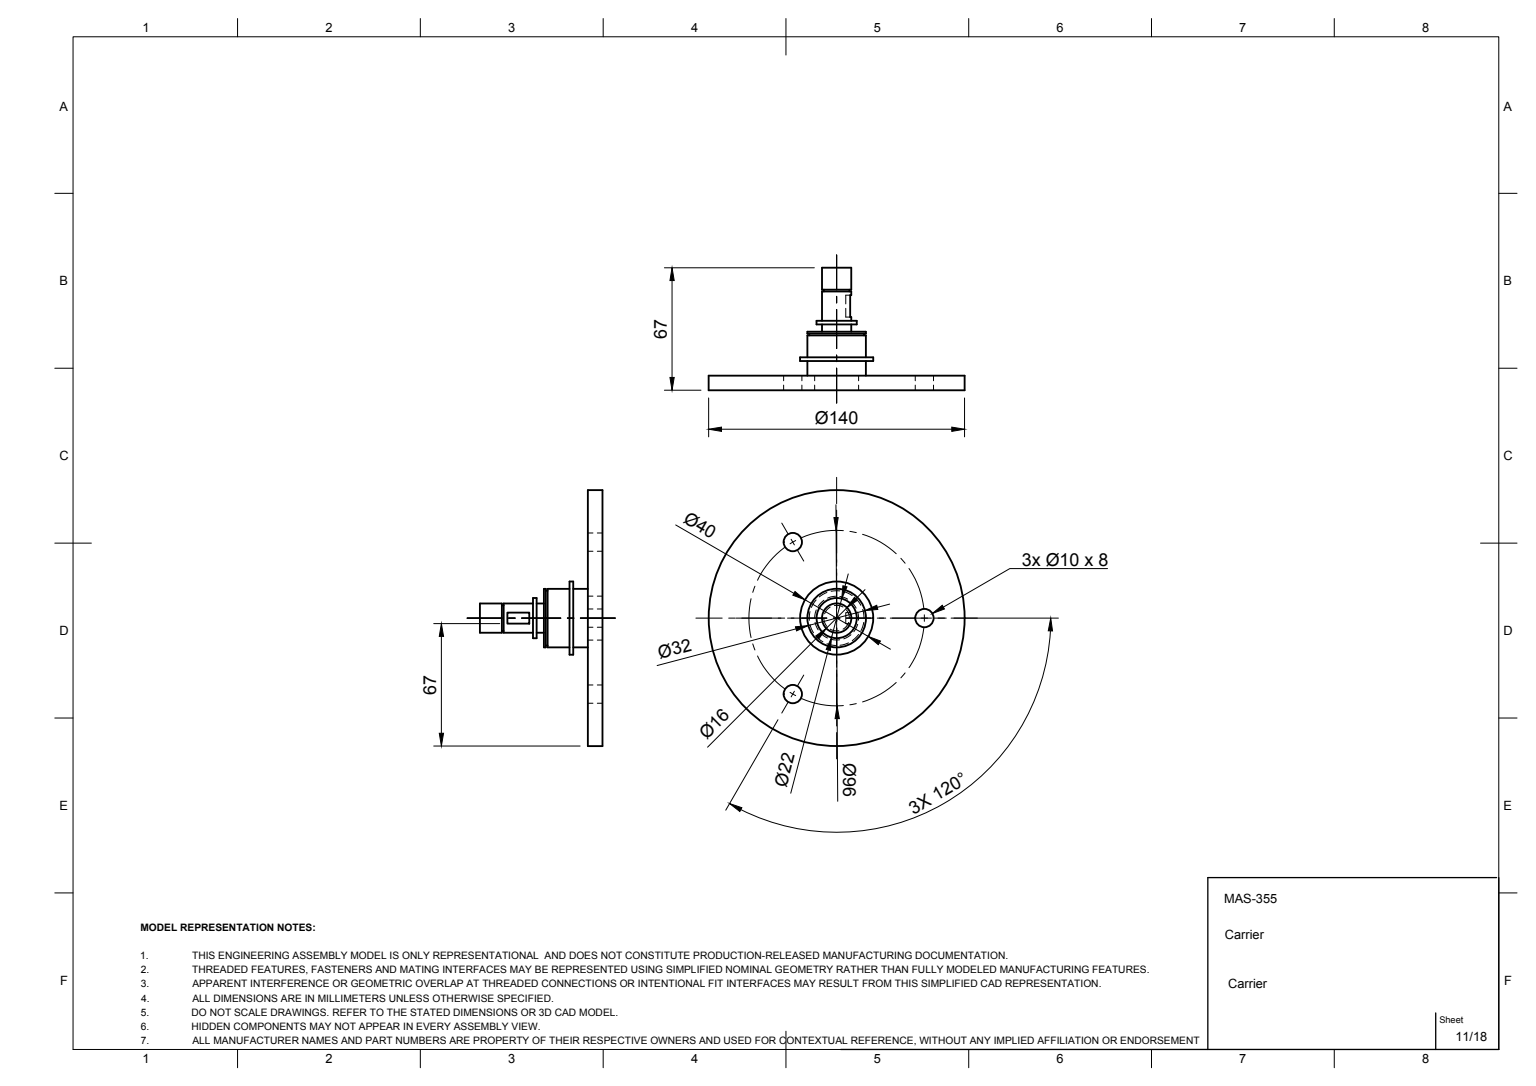
ISO-10303-21;
HEADER;
/* Generated by software containing ST-Developer
 * from STEP Tools, Inc. (www.steptools.com) 
 */

FILE_DESCRIPTION(
/* description */ ('Independent two-stage fixed-ring planetary gearbox,24/24/72 teeth,mod
ule2,20deg involutes,three planets per stage,4:1 x4:1=16:1. Native cut
-space/fillet/pattern tooth profiles derived from reusable gear blanks
; shared sun/planet/ring/carrier parts across both stages. Captured br
onze-journal input/carriers, headed retained planet pins, keyed inters
tage drive and modular keyed output interface. Native ideal gear links
; no torque, precision grade, production backlash/fits, lubrication, s
peed or life rating.'),
/* implementation_level */ '2;1');

FILE_NAME(
/* name */ 'Carrier.step',
/* time_stamp */ '2026-11-08T19:10:00-08:00',
/* author */ (''),
/* organization */ (''),
/* preprocessor_version */ 'ST-DEVELOPER v20.2',
/* originating_system */ 'Autodesk Translation Framework v15.17.0.0',
/* authorisation */ '');

FILE_SCHEMA (('AUTOMOTIVE_DESIGN { 1 0 10303 214 3 1 1 }'));
ENDSEC;

DATA;
#10=MECHANICAL_DESIGN_GEOMETRIC_PRESENTATION_REPRESENTATION('',(#1171),#259224);
#1131=SHAPE_REPRESENTATION_RELATIONSHIP('SRR','None',#259378,#1151);
#1151=ADVANCED_BREP_SHAPE_REPRESENTATION('',(#1191),#259212);
#1171=STYLED_ITEM('',(#259486),#1191);
#1191=MANIFOLD_SOLID_BREP('Body1',#25158);
#1287=FACE_BOUND('',#4341,.T.);
#1288=FACE_BOUND('',#4343,.T.);
#1289=FACE_BOUND('',#4347,.T.);
#1290=FACE_BOUND('',#4349,.T.);
#1291=FACE_BOUND('',#4355,.T.);
#1292=FACE_BOUND('',#4357,.T.);
#1293=FACE_BOUND('',#4361,.T.);
#1294=FACE_BOUND('',#4364,.T.);
#1295=FACE_BOUND('',#4366,.T.);
#1296=FACE_BOUND('',#4372,.T.);
#1297=FACE_BOUND('',#4376,.T.);
#1298=FACE_BOUND('',#4377,.T.);
#1299=FACE_BOUND('',#4378,.T.);
#1300=FACE_BOUND('',#4379,.T.);
#1301=FACE_BOUND('',#4381,.T.);
#1302=FACE_BOUND('',#4382,.T.);
#1303=FACE_BOUND('',#4383,.T.);
#1304=FACE_BOUND('',#4384,.T.);
#1637=PLANE('',#27011);
#1638=PLANE('',#27012);
#1639=PLANE('',#27014);
#1640=PLANE('',#27015);
#1641=PLANE('',#27016);
#1642=PLANE('',#27021);
#1643=PLANE('',#27023);
#1644=PLANE('',#27030);
#1645=PLANE('',#27032);
#1646=PLANE('',#27045);
#1647=PLANE('',#27048);
#1648=PLANE('',#27055);
#1649=PLANE('',#27056);
#1650=PLANE('',#27059);
#1651=PLANE('',#27065);
#1652=PLANE('',#27068);
#1653=PLANE('',#27074);
#1654=PLANE('',#27075);
#2904=FACE_OUTER_BOUND('',#4334,.T.);
#2905=FACE_OUTER_BOUND('',#4335,.T.);
#2906=FACE_OUTER_BOUND('',#4336,.T.);
#2907=FACE_OUTER_BOUND('',#4337,.T.);
#2908=FACE_OUTER_BOUND('',#4338,.T.);
#2909=FACE_OUTER_BOUND('',#4339,.T.);
#2910=FACE_OUTER_BOUND('',#4340,.T.);
#2911=FACE_OUTER_BOUND('',#4342,.T.);
#2912=FACE_OUTER_BOUND('',#4344,.T.);
#2913=FACE_OUTER_BOUND('',#4345,.T.);
#2914=FACE_OUTER_BOUND('',#4346,.T.);
#2915=FACE_OUTER_BOUND('',#4348,.T.);
#2916=FACE_OUTER_BOUND('',#4350,.T.);
#2917=FACE_OUTER_BOUND('',#4351,.T.);
#2918=FACE_OUTER_BOUND('',#4352,.T.);
#2919=FACE_OUTER_BOUND('',#4353,.T.);
#2920=FACE_OUTER_BOUND('',#4354,.T.);
#2921=FACE_OUTER_BOUND('',#4356,.T.);
#2922=FACE_OUTER_BOUND('',#4358,.T.);
#2923=FACE_OUTER_BOUND('',#4359,.T.);
#2924=FACE_OUTER_BOUND('',#4360,.T.);
#2925=FACE_OUTER_BOUND('',#4362,.T.);
#2926=FACE_OUTER_BOUND('',#4363,.T.);
#2927=FACE_OUTER_BOUND('',#4365,.T.);
#2928=FACE_OUTER_BOUND('',#4367,.T.);
#2929=FACE_OUTER_BOUND('',#4368,.T.);
#2930=FACE_OUTER_BOUND('',#4369,.T.);
#2931=FACE_OUTER_BOUND('',#4370,.T.);
#2932=FACE_OUTER_BOUND('',#4371,.T.);
#2933=FACE_OUTER_BOUND('',#4373,.T.);
#2934=FACE_OUTER_BOUND('',#4374,.T.);
#2935=FACE_OUTER_BOUND('',#4375,.T.);
#2936=FACE_OUTER_BOUND('',#4380,.T.);
#4334=EDGE_LOOP('',(#22484,#22485,#22486,#22487));
#4335=EDGE_LOOP('',(#22488,#22489,#22490,#22491));
#4336=EDGE_LOOP('',(#22492,#22493,#22494,#22495));
#4337=EDGE_LOOP('',(#22496,#22497,#22498,#22499));
#4338=EDGE_LOOP('',(#22500,#22501,#22502,#22503));
#4339=EDGE_LOOP('',(#22504,#22505,#22506,#22507));
#4340=EDGE_LOOP('',(#22508));
#4341=EDGE_LOOP('',(#22509));
#4342=EDGE_LOOP('',(#22510));
#4343=EDGE_LOOP('',(#22511));
#4344=EDGE_LOOP('',(#22512,#22513,#22514,#22515));
#4345=EDGE_LOOP('',(#22516,#22517,#22518,#22519));
#4346=EDGE_LOOP('',(#22520));
#4347=EDGE_LOOP('',(#22521));
#4348=EDGE_LOOP('',(#22522));
#4349=EDGE_LOOP('',(#22523));
#4350=EDGE_LOOP('',(#22524,#22525,#22526,#22527));
#4351=EDGE_LOOP('',(#22528,#22529,#22530,#22531));
#4352=EDGE_LOOP('',(#22532,#22533,#22534,#22535));
#4353=EDGE_LOOP('',(#22536,#22537,#22538,#22539));
#4354=EDGE_LOOP('',(#22540));
#4355=EDGE_LOOP('',(#22541));
#4356=EDGE_LOOP('',(#22542));
#4357=EDGE_LOOP('',(#22543));
#4358=EDGE_LOOP('',(#22544,#22545,#22546,#22547));
#4359=EDGE_LOOP('',(#22548,#22549,#22550,#22551));
#4360=EDGE_LOOP('',(#22552,#22553,#22554,#22555));
#4361=EDGE_LOOP('',(#22556,#22557,#22558,#22559));
#4362=EDGE_LOOP('',(#22560));
#4363=EDGE_LOOP('',(#22561));
#4364=EDGE_LOOP('',(#22562));
#4365=EDGE_LOOP('',(#22563));
#4366=EDGE_LOOP('',(#22564));
#4367=EDGE_LOOP('',(#22565,#22566,#22567,#22568));
#4368=EDGE_LOOP('',(#22569,#22570,#22571,#22572));
#4369=EDGE_LOOP('',(#22573));
#4370=EDGE_LOOP('',(#22574,#22575,#22576,#22577));
#4371=EDGE_LOOP('',(#22578));
#4372=EDGE_LOOP('',(#22579));
#4373=EDGE_LOOP('',(#22580,#22581,#22582,#22583));
#4374=EDGE_LOOP('',(#22584,#22585,#22586,#22587));
#4375=EDGE_LOOP('',(#22588));
#4376=EDGE_LOOP('',(#22589));
#4377=EDGE_LOOP('',(#22590));
#4378=EDGE_LOOP('',(#22591));
#4379=EDGE_LOOP('',(#22592));
#4380=EDGE_LOOP('',(#22593));
#4381=EDGE_LOOP('',(#22594));
#4382=EDGE_LOOP('',(#22595));
#4383=EDGE_LOOP('',(#22596));
#4384=EDGE_LOOP('',(#22597));
#5309=CIRCLE('',#27013,8.);
#5310=CIRCLE('',#27017,8.);
#5311=CIRCLE('',#27019,7.);
#5312=CIRCLE('',#27020,7.);
#5313=CIRCLE('',#27022,8.);
#5314=CIRCLE('',#27024,8.);
#5315=CIRCLE('',#27026,8.);
#5316=CIRCLE('',#27028,15.);
#5317=CIRCLE('',#27029,15.);
#5318=CIRCLE('',#27031,16.);
#5319=CIRCLE('',#27033,16.);
#5320=CIRCLE('',#27035,16.);
#5321=CIRCLE('',#27037,5.);
#5322=CIRCLE('',#27038,5.);
#5323=CIRCLE('',#27040,5.);
#5324=CIRCLE('',#27041,5.);
#5325=CIRCLE('',#27043,5.);
#5326=CIRCLE('',#27044,5.);
#5327=CIRCLE('',#27046,11.);
#5328=CIRCLE('',#27047,8.);
#5329=CIRCLE('',#27049,11.);
#5330=CIRCLE('',#27050,8.);
#5331=CIRCLE('',#27053,8.);
#5332=CIRCLE('',#27057,20.);
#5333=CIRCLE('',#27058,16.);
#5334=CIRCLE('',#27060,20.);
#5335=CIRCLE('',#27061,16.);
#5336=CIRCLE('',#27064,16.);
#5337=CIRCLE('',#27066,12.);
#5338=CIRCLE('',#27070,12.);
#5339=CIRCLE('',#27072,70.);
#5340=CIRCLE('',#27073,70.);
#7719=LINE('',#255776,#8904);
#7720=LINE('',#255778,#8905);
#7721=LINE('',#255780,#8906);
#7722=LINE('',#255781,#8907);
#7723=LINE('',#255786,#8908);
#7724=LINE('',#255787,#8909);
#7725=LINE('',#255790,#8910);
#7726=LINE('',#255792,#8911);
#7727=LINE('',#255793,#8912);
#7728=LINE('',#255795,#8913);
#7729=LINE('',#255802,#8914);
#7730=LINE('',#255813,#8915);
#7731=LINE('',#255818,#8916);
#7732=LINE('',#255829,#8917);
#7733=LINE('',#255834,#8918);
#7734=LINE('',#255840,#8919);
#7735=LINE('',#255846,#8920);
#7736=LINE('',#255859,#8921);
#7737=LINE('',#255862,#8922);
#7738=LINE('',#255865,#8923);
#7739=LINE('',#255878,#8924);
#7740=LINE('',#255881,#8925);
#7741=LINE('',#255887,#8926);
#7742=LINE('',#255891,#8927);
#7743=LINE('',#255897,#8928);
#8904=VECTOR('',#31628,10.);
#8905=VECTOR('',#31629,10.);
#8906=VECTOR('',#31630,10.);
#8907=VECTOR('',#31631,10.);
#8908=VECTOR('',#31636,10.);
#8909=VECTOR('',#31637,10.);
#8910=VECTOR('',#31640,10.);
#8911=VECTOR('',#31641,10.);
#8912=VECTOR('',#31642,10.);
#8913=VECTOR('',#31645,10.);
#8914=VECTOR('',#31654,7.);
#8915=VECTOR('',#31669,8.);
#8916=VECTOR('',#31674,15.);
#8917=VECTOR('',#31689,16.);
#8918=VECTOR('',#31694,5.);
#8919=VECTOR('',#31701,5.);
#8920=VECTOR('',#31708,5.);
#8921=VECTOR('',#31725,11.);
#8922=VECTOR('',#31728,8.);
#8923=VECTOR('',#31733,8.);
#8924=VECTOR('',#31750,20.);
#8925=VECTOR('',#31753,16.);
#8926=VECTOR('',#31762,16.);
#8927=VECTOR('',#31767,12.);
#8928=VECTOR('',#31774,70.);
#11399=VERTEX_POINT('',#255774);
#11400=VERTEX_POINT('',#255775);
#11401=VERTEX_POINT('',#255777);
#11402=VERTEX_POINT('',#255779);
#11403=VERTEX_POINT('',#255783);
#11404=VERTEX_POINT('',#255785);
#11405=VERTEX_POINT('',#255789);
#11406=VERTEX_POINT('',#255791);
#11407=VERTEX_POINT('',#255799);
#11408=VERTEX_POINT('',#255801);
#11409=VERTEX_POINT('',#255805);
#11410=VERTEX_POINT('',#255808);
#11411=VERTEX_POINT('',#255811);
#11412=VERTEX_POINT('',#255815);
#11413=VERTEX_POINT('',#255817);
#11414=VERTEX_POINT('',#255821);
#11415=VERTEX_POINT('',#255824);
#11416=VERTEX_POINT('',#255827);
#11417=VERTEX_POINT('',#255831);
#11418=VERTEX_POINT('',#255833);
#11419=VERTEX_POINT('',#255837);
#11420=VERTEX_POINT('',#255839);
#11421=VERTEX_POINT('',#255843);
#11422=VERTEX_POINT('',#255845);
#11423=VERTEX_POINT('',#255849);
#11424=VERTEX_POINT('',#255851);
#11425=VERTEX_POINT('',#255854);
#11426=VERTEX_POINT('',#255856);
#11427=VERTEX_POINT('',#255861);
#11428=VERTEX_POINT('',#255868);
#11429=VERTEX_POINT('',#255870);
#11430=VERTEX_POINT('',#255873);
#11431=VERTEX_POINT('',#255875);
#11432=VERTEX_POINT('',#255880);
#11433=VERTEX_POINT('',#255884);
#11434=VERTEX_POINT('',#255890);
#11435=VERTEX_POINT('',#255894);
#11436=VERTEX_POINT('',#255896);
#15127=EDGE_CURVE('',#11399,#11400,#7719,.T.);
#15128=EDGE_CURVE('',#11399,#11401,#7720,.T.);
#15129=EDGE_CURVE('',#11402,#11401,#7721,.T.);
#15130=EDGE_CURVE('',#11402,#11400,#7722,.T.);
#15131=EDGE_CURVE('',#11400,#11403,#5309,.T.);
#15132=EDGE_CURVE('',#11404,#11402,#7723,.T.);
#15133=EDGE_CURVE('',#11403,#11404,#7724,.T.);
#15134=EDGE_CURVE('',#11403,#11405,#7725,.T.);
#15135=EDGE_CURVE('',#11404,#11406,#7726,.T.);
#15136=EDGE_CURVE('',#11406,#11405,#7727,.T.);
#15137=EDGE_CURVE('',#11401,#11406,#7728,.T.);
#15138=EDGE_CURVE('',#11405,#11399,#5310,.T.);
#15139=EDGE_CURVE('',#11407,#11407,#5311,.T.);
#15140=EDGE_CURVE('',#11407,#11408,#7729,.T.);
#15141=EDGE_CURVE('',#11408,#11408,#5312,.T.);
#15142=EDGE_CURVE('',#11409,#11409,#5313,.T.);
#15143=EDGE_CURVE('',#11410,#11410,#5314,.T.);
#15144=EDGE_CURVE('',#11411,#11411,#5315,.T.);
#15145=EDGE_CURVE('',#11411,#11410,#7730,.T.);
#15146=EDGE_CURVE('',#11412,#11412,#5316,.T.);
#15147=EDGE_CURVE('',#11412,#11413,#7731,.T.);
#15148=EDGE_CURVE('',#11413,#11413,#5317,.T.);
#15149=EDGE_CURVE('',#11414,#11414,#5318,.T.);
#15150=EDGE_CURVE('',#11415,#11415,#5319,.T.);
#15151=EDGE_CURVE('',#11416,#11416,#5320,.T.);
#15152=EDGE_CURVE('',#11416,#11415,#7732,.T.);
#15153=EDGE_CURVE('',#11417,#11417,#5321,.T.);
#15154=EDGE_CURVE('',#11417,#11418,#7733,.T.);
#15155=EDGE_CURVE('',#11418,#11418,#5322,.T.);
#15156=EDGE_CURVE('',#11419,#11419,#5323,.T.);
#15157=EDGE_CURVE('',#11419,#11420,#7734,.T.);
#15158=EDGE_CURVE('',#11420,#11420,#5324,.T.);
#15159=EDGE_CURVE('',#11421,#11421,#5325,.T.);
#15160=EDGE_CURVE('',#11421,#11422,#7735,.T.);
#15161=EDGE_CURVE('',#11422,#11422,#5326,.T.);
#15162=EDGE_CURVE('',#11423,#11423,#5327,.T.);
#15163=EDGE_CURVE('',#11424,#11424,#5328,.T.);
#15164=EDGE_CURVE('',#11425,#11425,#5329,.T.);
#15165=EDGE_CURVE('',#11426,#11426,#5330,.T.);
#15166=EDGE_CURVE('',#11423,#11425,#7736,.T.);
#15167=EDGE_CURVE('',#11426,#11427,#7737,.T.);
#15168=EDGE_CURVE('',#11427,#11427,#5331,.T.);
#15169=EDGE_CURVE('',#11409,#11424,#7738,.T.);
#15170=EDGE_CURVE('',#11428,#11428,#5332,.T.);
#15171=EDGE_CURVE('',#11429,#11429,#5333,.T.);
#15172=EDGE_CURVE('',#11430,#11430,#5334,.T.);
#15173=EDGE_CURVE('',#11431,#11431,#5335,.T.);
#15174=EDGE_CURVE('',#11428,#11430,#7739,.T.);
#15175=EDGE_CURVE('',#11431,#11432,#7740,.T.);
#15176=EDGE_CURVE('',#11432,#11432,#5336,.T.);
#15177=EDGE_CURVE('',#11433,#11433,#5337,.T.);
#15178=EDGE_CURVE('',#11414,#11429,#7741,.T.);
#15179=EDGE_CURVE('',#11433,#11434,#7742,.T.);
#15180=EDGE_CURVE('',#11434,#11434,#5338,.T.);
#15181=EDGE_CURVE('',#11435,#11435,#5339,.T.);
#15182=EDGE_CURVE('',#11435,#11436,#7743,.T.);
#15183=EDGE_CURVE('',#11436,#11436,#5340,.T.);
#22484=ORIENTED_EDGE('',*,*,#15127,.F.);
#22485=ORIENTED_EDGE('',*,*,#15128,.T.);
#22486=ORIENTED_EDGE('',*,*,#15129,.F.);
#22487=ORIENTED_EDGE('',*,*,#15130,.T.);
#22488=ORIENTED_EDGE('',*,*,#15131,.F.);
#22489=ORIENTED_EDGE('',*,*,#15130,.F.);
#22490=ORIENTED_EDGE('',*,*,#15132,.F.);
#22491=ORIENTED_EDGE('',*,*,#15133,.F.);
#22492=ORIENTED_EDGE('',*,*,#15134,.F.);
#22493=ORIENTED_EDGE('',*,*,#15133,.T.);
#22494=ORIENTED_EDGE('',*,*,#15135,.T.);
#22495=ORIENTED_EDGE('',*,*,#15136,.T.);
#22496=ORIENTED_EDGE('',*,*,#15132,.T.);
#22497=ORIENTED_EDGE('',*,*,#15129,.T.);
#22498=ORIENTED_EDGE('',*,*,#15137,.T.);
#22499=ORIENTED_EDGE('',*,*,#15135,.F.);
#22500=ORIENTED_EDGE('',*,*,#15138,.F.);
#22501=ORIENTED_EDGE('',*,*,#15136,.F.);
#22502=ORIENTED_EDGE('',*,*,#15137,.F.);
#22503=ORIENTED_EDGE('',*,*,#15128,.F.);
#22504=ORIENTED_EDGE('',*,*,#15139,.T.);
#22505=ORIENTED_EDGE('',*,*,#15140,.T.);
#22506=ORIENTED_EDGE('',*,*,#15141,.F.);
#22507=ORIENTED_EDGE('',*,*,#15140,.F.);
#22508=ORIENTED_EDGE('',*,*,#15142,.F.);
#22509=ORIENTED_EDGE('',*,*,#15139,.F.);
#22510=ORIENTED_EDGE('',*,*,#15143,.F.);
#22511=ORIENTED_EDGE('',*,*,#15141,.T.);
#22512=ORIENTED_EDGE('',*,*,#15144,.F.);
#22513=ORIENTED_EDGE('',*,*,#15145,.T.);
#22514=ORIENTED_EDGE('',*,*,#15143,.T.);
#22515=ORIENTED_EDGE('',*,*,#15145,.F.);
#22516=ORIENTED_EDGE('',*,*,#15146,.T.);
#22517=ORIENTED_EDGE('',*,*,#15147,.T.);
#22518=ORIENTED_EDGE('',*,*,#15148,.F.);
#22519=ORIENTED_EDGE('',*,*,#15147,.F.);
#22520=ORIENTED_EDGE('',*,*,#15149,.F.);
#22521=ORIENTED_EDGE('',*,*,#15146,.F.);
#22522=ORIENTED_EDGE('',*,*,#15150,.F.);
#22523=ORIENTED_EDGE('',*,*,#15148,.T.);
#22524=ORIENTED_EDGE('',*,*,#15151,.F.);
#22525=ORIENTED_EDGE('',*,*,#15152,.T.);
#22526=ORIENTED_EDGE('',*,*,#15150,.T.);
#22527=ORIENTED_EDGE('',*,*,#15152,.F.);
#22528=ORIENTED_EDGE('',*,*,#15153,.F.);
#22529=ORIENTED_EDGE('',*,*,#15154,.T.);
#22530=ORIENTED_EDGE('',*,*,#15155,.F.);
#22531=ORIENTED_EDGE('',*,*,#15154,.F.);
#22532=ORIENTED_EDGE('',*,*,#15156,.F.);
#22533=ORIENTED_EDGE('',*,*,#15157,.T.);
#22534=ORIENTED_EDGE('',*,*,#15158,.F.);
#22535=ORIENTED_EDGE('',*,*,#15157,.F.);
#22536=ORIENTED_EDGE('',*,*,#15159,.F.);
#22537=ORIENTED_EDGE('',*,*,#15160,.T.);
#22538=ORIENTED_EDGE('',*,*,#15161,.F.);
#22539=ORIENTED_EDGE('',*,*,#15160,.F.);
#22540=ORIENTED_EDGE('',*,*,#15162,.T.);
#22541=ORIENTED_EDGE('',*,*,#15163,.F.);
#22542=ORIENTED_EDGE('',*,*,#15164,.F.);
#22543=ORIENTED_EDGE('',*,*,#15165,.F.);
#22544=ORIENTED_EDGE('',*,*,#15162,.F.);
#22545=ORIENTED_EDGE('',*,*,#15166,.T.);
#22546=ORIENTED_EDGE('',*,*,#15164,.T.);
#22547=ORIENTED_EDGE('',*,*,#15166,.F.);
#22548=ORIENTED_EDGE('',*,*,#15165,.T.);
#22549=ORIENTED_EDGE('',*,*,#15167,.T.);
#22550=ORIENTED_EDGE('',*,*,#15168,.F.);
#22551=ORIENTED_EDGE('',*,*,#15167,.F.);
#22552=ORIENTED_EDGE('',*,*,#15142,.T.);
#22553=ORIENTED_EDGE('',*,*,#15169,.T.);
#22554=ORIENTED_EDGE('',*,*,#15163,.T.);
#22555=ORIENTED_EDGE('',*,*,#15169,.F.);
#22556=ORIENTED_EDGE('',*,*,#15134,.T.);
#22557=ORIENTED_EDGE('',*,*,#15138,.T.);
#22558=ORIENTED_EDGE('',*,*,#15127,.T.);
#22559=ORIENTED_EDGE('',*,*,#15131,.T.);
#22560=ORIENTED_EDGE('',*,*,#15144,.T.);
#22561=ORIENTED_EDGE('',*,*,#15170,.T.);
#22562=ORIENTED_EDGE('',*,*,#15171,.F.);
#22563=ORIENTED_EDGE('',*,*,#15172,.F.);
#22564=ORIENTED_EDGE('',*,*,#15173,.F.);
#22565=ORIENTED_EDGE('',*,*,#15170,.F.);
#22566=ORIENTED_EDGE('',*,*,#15174,.T.);
#22567=ORIENTED_EDGE('',*,*,#15172,.T.);
#22568=ORIENTED_EDGE('',*,*,#15174,.F.);
#22569=ORIENTED_EDGE('',*,*,#15173,.T.);
#22570=ORIENTED_EDGE('',*,*,#15175,.T.);
#22571=ORIENTED_EDGE('',*,*,#15176,.F.);
#22572=ORIENTED_EDGE('',*,*,#15175,.F.);
#22573=ORIENTED_EDGE('',*,*,#15177,.T.);
#22574=ORIENTED_EDGE('',*,*,#15149,.T.);
#22575=ORIENTED_EDGE('',*,*,#15178,.T.);
#22576=ORIENTED_EDGE('',*,*,#15171,.T.);
#22577=ORIENTED_EDGE('',*,*,#15178,.F.);
#22578=ORIENTED_EDGE('',*,*,#15151,.T.);
#22579=ORIENTED_EDGE('',*,*,#15168,.T.);
#22580=ORIENTED_EDGE('',*,*,#15177,.F.);
#22581=ORIENTED_EDGE('',*,*,#15179,.T.);
#22582=ORIENTED_EDGE('',*,*,#15180,.T.);
#22583=ORIENTED_EDGE('',*,*,#15179,.F.);
#22584=ORIENTED_EDGE('',*,*,#15181,.F.);
#22585=ORIENTED_EDGE('',*,*,#15182,.T.);
#22586=ORIENTED_EDGE('',*,*,#15183,.T.);
#22587=ORIENTED_EDGE('',*,*,#15182,.F.);
#22588=ORIENTED_EDGE('',*,*,#15181,.T.);
#22589=ORIENTED_EDGE('',*,*,#15153,.T.);
#22590=ORIENTED_EDGE('',*,*,#15156,.T.);
#22591=ORIENTED_EDGE('',*,*,#15159,.T.);
#22592=ORIENTED_EDGE('',*,*,#15176,.T.);
#22593=ORIENTED_EDGE('',*,*,#15183,.F.);
#22594=ORIENTED_EDGE('',*,*,#15155,.T.);
#22595=ORIENTED_EDGE('',*,*,#15158,.T.);
#22596=ORIENTED_EDGE('',*,*,#15161,.T.);
#22597=ORIENTED_EDGE('',*,*,#15180,.F.);
#23727=CYLINDRICAL_SURFACE('',#27018,7.);
#23728=CYLINDRICAL_SURFACE('',#27025,8.);
#23729=CYLINDRICAL_SURFACE('',#27027,15.);
#23730=CYLINDRICAL_SURFACE('',#27034,16.);
#23731=CYLINDRICAL_SURFACE('',#27036,5.);
#23732=CYLINDRICAL_SURFACE('',#27039,5.);
#23733=CYLINDRICAL_SURFACE('',#27042,5.);
#23734=CYLINDRICAL_SURFACE('',#27051,11.);
#23735=CYLINDRICAL_SURFACE('',#27052,8.);
#23736=CYLINDRICAL_SURFACE('',#27054,8.);
#23737=CYLINDRICAL_SURFACE('',#27062,20.);
#23738=CYLINDRICAL_SURFACE('',#27063,16.);
#23739=CYLINDRICAL_SURFACE('',#27067,16.);
#23740=CYLINDRICAL_SURFACE('',#27069,12.);
#23741=CYLINDRICAL_SURFACE('',#27071,70.);
#25010=ADVANCED_FACE('',(#2904),#1637,.F.);
#25011=ADVANCED_FACE('',(#2905),#1638,.F.);
#25012=ADVANCED_FACE('',(#2906),#1639,.F.);
#25013=ADVANCED_FACE('',(#2907),#1640,.F.);
#25014=ADVANCED_FACE('',(#2908),#1641,.F.);
#25015=ADVANCED_FACE('',(#2909),#23727,.T.);
#25016=ADVANCED_FACE('',(#2910,#1287),#1642,.F.);
#25017=ADVANCED_FACE('',(#2911,#1288),#1643,.F.);
#25018=ADVANCED_FACE('',(#2912),#23728,.T.);
#25019=ADVANCED_FACE('',(#2913),#23729,.T.);
#25020=ADVANCED_FACE('',(#2914,#1289),#1644,.F.);
#25021=ADVANCED_FACE('',(#2915,#1290),#1645,.F.);
#25022=ADVANCED_FACE('',(#2916),#23730,.T.);
#25023=ADVANCED_FACE('',(#2917),#23731,.F.);
#25024=ADVANCED_FACE('',(#2918),#23732,.F.);
#25025=ADVANCED_FACE('',(#2919),#23733,.F.);
#25026=ADVANCED_FACE('',(#2920,#1291),#1646,.T.);
#25027=ADVANCED_FACE('',(#2921,#1292),#1647,.F.);
#25028=ADVANCED_FACE('',(#2922),#23734,.T.);
#25029=ADVANCED_FACE('',(#2923),#23735,.T.);
#25030=ADVANCED_FACE('',(#2924,#1293),#23736,.T.);
#25031=ADVANCED_FACE('',(#2925),#1648,.T.);
#25032=ADVANCED_FACE('',(#2926,#1294),#1649,.T.);
#25033=ADVANCED_FACE('',(#2927,#1295),#1650,.F.);
#25034=ADVANCED_FACE('',(#2928),#23737,.T.);
#25035=ADVANCED_FACE('',(#2929),#23738,.T.);
#25036=ADVANCED_FACE('',(#2930),#1651,.F.);
#25037=ADVANCED_FACE('',(#2931),#23739,.T.);
#25038=ADVANCED_FACE('',(#2932,#1296),#1652,.T.);
#25039=ADVANCED_FACE('',(#2933),#23740,.F.);
#25040=ADVANCED_FACE('',(#2934),#23741,.T.);
#25041=ADVANCED_FACE('',(#2935,#1297,#1298,#1299,#1300),#1653,.T.);
#25042=ADVANCED_FACE('',(#2936,#1301,#1302,#1303,#1304),#1654,.F.);
#25158=CLOSED_SHELL('',(#25010,#25011,#25012,#25013,#25014,#25015,#25016,
#25017,#25018,#25019,#25020,#25021,#25022,#25023,#25024,#25025,#25026,#25027,
#25028,#25029,#25030,#25031,#25032,#25033,#25034,#25035,#25036,#25037,#25038,
#25039,#25040,#25041,#25042));
#27010=AXIS2_PLACEMENT_3D('',#255772,#31624,#31625);
#27011=AXIS2_PLACEMENT_3D('',#255773,#31626,#31627);
#27012=AXIS2_PLACEMENT_3D('',#255782,#31632,#31633);
#27013=AXIS2_PLACEMENT_3D('',#255784,#31634,#31635);
#27014=AXIS2_PLACEMENT_3D('',#255788,#31638,#31639);
#27015=AXIS2_PLACEMENT_3D('',#255794,#31643,#31644);
#27016=AXIS2_PLACEMENT_3D('',#255796,#31646,#31647);
#27017=AXIS2_PLACEMENT_3D('',#255797,#31648,#31649);
#27018=AXIS2_PLACEMENT_3D('',#255798,#31650,#31651);
#27019=AXIS2_PLACEMENT_3D('',#255800,#31652,#31653);
#27020=AXIS2_PLACEMENT_3D('',#255803,#31655,#31656);
#27021=AXIS2_PLACEMENT_3D('',#255804,#31657,#31658);
#27022=AXIS2_PLACEMENT_3D('',#255806,#31659,#31660);
#27023=AXIS2_PLACEMENT_3D('',#255807,#31661,#31662);
#27024=AXIS2_PLACEMENT_3D('',#255809,#31663,#31664);
#27025=AXIS2_PLACEMENT_3D('',#255810,#31665,#31666);
#27026=AXIS2_PLACEMENT_3D('',#255812,#31667,#31668);
#27027=AXIS2_PLACEMENT_3D('',#255814,#31670,#31671);
#27028=AXIS2_PLACEMENT_3D('',#255816,#31672,#31673);
#27029=AXIS2_PLACEMENT_3D('',#255819,#31675,#31676);
#27030=AXIS2_PLACEMENT_3D('',#255820,#31677,#31678);
#27031=AXIS2_PLACEMENT_3D('',#255822,#31679,#31680);
#27032=AXIS2_PLACEMENT_3D('',#255823,#31681,#31682);
#27033=AXIS2_PLACEMENT_3D('',#255825,#31683,#31684);
#27034=AXIS2_PLACEMENT_3D('',#255826,#31685,#31686);
#27035=AXIS2_PLACEMENT_3D('',#255828,#31687,#31688);
#27036=AXIS2_PLACEMENT_3D('',#255830,#31690,#31691);
#27037=AXIS2_PLACEMENT_3D('',#255832,#31692,#31693);
#27038=AXIS2_PLACEMENT_3D('',#255835,#31695,#31696);
#27039=AXIS2_PLACEMENT_3D('',#255836,#31697,#31698);
#27040=AXIS2_PLACEMENT_3D('',#255838,#31699,#31700);
#27041=AXIS2_PLACEMENT_3D('',#255841,#31702,#31703);
#27042=AXIS2_PLACEMENT_3D('',#255842,#31704,#31705);
#27043=AXIS2_PLACEMENT_3D('',#255844,#31706,#31707);
#27044=AXIS2_PLACEMENT_3D('',#255847,#31709,#31710);
#27045=AXIS2_PLACEMENT_3D('',#255848,#31711,#31712);
#27046=AXIS2_PLACEMENT_3D('',#255850,#31713,#31714);
#27047=AXIS2_PLACEMENT_3D('',#255852,#31715,#31716);
#27048=AXIS2_PLACEMENT_3D('',#255853,#31717,#31718);
#27049=AXIS2_PLACEMENT_3D('',#255855,#31719,#31720);
#27050=AXIS2_PLACEMENT_3D('',#255857,#31721,#31722);
#27051=AXIS2_PLACEMENT_3D('',#255858,#31723,#31724);
#27052=AXIS2_PLACEMENT_3D('',#255860,#31726,#31727);
#27053=AXIS2_PLACEMENT_3D('',#255863,#31729,#31730);
#27054=AXIS2_PLACEMENT_3D('',#255864,#31731,#31732);
#27055=AXIS2_PLACEMENT_3D('',#255866,#31734,#31735);
#27056=AXIS2_PLACEMENT_3D('',#255867,#31736,#31737);
#27057=AXIS2_PLACEMENT_3D('',#255869,#31738,#31739);
#27058=AXIS2_PLACEMENT_3D('',#255871,#31740,#31741);
#27059=AXIS2_PLACEMENT_3D('',#255872,#31742,#31743);
#27060=AXIS2_PLACEMENT_3D('',#255874,#31744,#31745);
#27061=AXIS2_PLACEMENT_3D('',#255876,#31746,#31747);
#27062=AXIS2_PLACEMENT_3D('',#255877,#31748,#31749);
#27063=AXIS2_PLACEMENT_3D('',#255879,#31751,#31752);
#27064=AXIS2_PLACEMENT_3D('',#255882,#31754,#31755);
#27065=AXIS2_PLACEMENT_3D('',#255883,#31756,#31757);
#27066=AXIS2_PLACEMENT_3D('',#255885,#31758,#31759);
#27067=AXIS2_PLACEMENT_3D('',#255886,#31760,#31761);
#27068=AXIS2_PLACEMENT_3D('',#255888,#31763,#31764);
#27069=AXIS2_PLACEMENT_3D('',#255889,#31765,#31766);
#27070=AXIS2_PLACEMENT_3D('',#255892,#31768,#31769);
#27071=AXIS2_PLACEMENT_3D('',#255893,#31770,#31771);
#27072=AXIS2_PLACEMENT_3D('',#255895,#31772,#31773);
#27073=AXIS2_PLACEMENT_3D('',#255898,#31775,#31776);
#27074=AXIS2_PLACEMENT_3D('',#255899,#31777,#31778);
#27075=AXIS2_PLACEMENT_3D('',#255900,#31779,#31780);
#31624=DIRECTION('axis',(0.,0.,1.));
#31625=DIRECTION('refdir',(1.,0.,0.));
#31626=DIRECTION('center_axis',(0.,-1.,0.));
#31627=DIRECTION('ref_axis',(-1.,0.,0.));
#31628=DIRECTION('',(0.,0.,1.));
#31629=DIRECTION('',(-1.,0.,0.));
#31630=DIRECTION('',(0.,0.,-1.));
#31631=DIRECTION('',(1.,0.,0.));
#31632=DIRECTION('center_axis',(0.,0.,1.));
#31633=DIRECTION('ref_axis',(1.,0.,0.));
#31634=DIRECTION('center_axis',(0.,0.,1.));
#31635=DIRECTION('ref_axis',(1.,0.,0.));
#31636=DIRECTION('',(0.,-1.,0.));
#31637=DIRECTION('',(-1.,0.,0.));
#31638=DIRECTION('center_axis',(0.,1.,0.));
#31639=DIRECTION('ref_axis',(1.,0.,0.));
#31640=DIRECTION('',(0.,0.,-1.));
#31641=DIRECTION('',(0.,0.,-1.));
#31642=DIRECTION('',(1.,0.,0.));
#31643=DIRECTION('center_axis',(-1.,0.,0.));
#31644=DIRECTION('ref_axis',(0.,1.,0.));
#31645=DIRECTION('',(0.,1.,0.));
#31646=DIRECTION('center_axis',(0.,0.,-1.));
#31647=DIRECTION('ref_axis',(-1.,0.,0.));
#31648=DIRECTION('center_axis',(0.,0.,-1.));
#31649=DIRECTION('ref_axis',(1.,0.,0.));
#31650=DIRECTION('center_axis',(0.,0.,1.));
#31651=DIRECTION('ref_axis',(1.,0.,0.));
#31652=DIRECTION('center_axis',(0.,0.,1.));
#31653=DIRECTION('ref_axis',(1.,0.,0.));
#31654=DIRECTION('',(0.,0.,1.));
#31655=DIRECTION('center_axis',(0.,0.,1.));
#31656=DIRECTION('ref_axis',(1.,0.,0.));
#31657=DIRECTION('center_axis',(0.,0.,-1.));
#31658=DIRECTION('ref_axis',(-1.,0.,0.));
#31659=DIRECTION('center_axis',(0.,0.,-1.));
#31660=DIRECTION('ref_axis',(1.,0.,0.));
#31661=DIRECTION('center_axis',(0.,0.,1.));
#31662=DIRECTION('ref_axis',(1.,0.,0.));
#31663=DIRECTION('center_axis',(0.,0.,1.));
#31664=DIRECTION('ref_axis',(1.,0.,0.));
#31665=DIRECTION('center_axis',(0.,0.,1.));
#31666=DIRECTION('ref_axis',(1.,0.,0.));
#31667=DIRECTION('center_axis',(0.,0.,1.));
#31668=DIRECTION('ref_axis',(1.,0.,0.));
#31669=DIRECTION('',(0.,0.,-1.));
#31670=DIRECTION('center_axis',(0.,0.,1.));
#31671=DIRECTION('ref_axis',(1.,0.,0.));
#31672=DIRECTION('center_axis',(0.,0.,1.));
#31673=DIRECTION('ref_axis',(1.,0.,0.));
#31674=DIRECTION('',(0.,0.,1.));
#31675=DIRECTION('center_axis',(0.,0.,1.));
#31676=DIRECTION('ref_axis',(1.,0.,0.));
#31677=DIRECTION('center_axis',(0.,0.,-1.));
#31678=DIRECTION('ref_axis',(-1.,0.,0.));
#31679=DIRECTION('center_axis',(0.,0.,-1.));
#31680=DIRECTION('ref_axis',(1.,0.,0.));
#31681=DIRECTION('center_axis',(0.,0.,1.));
#31682=DIRECTION('ref_axis',(1.,0.,0.));
#31683=DIRECTION('center_axis',(0.,0.,1.));
#31684=DIRECTION('ref_axis',(1.,0.,0.));
#31685=DIRECTION('center_axis',(0.,0.,1.));
#31686=DIRECTION('ref_axis',(1.,0.,0.));
#31687=DIRECTION('center_axis',(0.,0.,1.));
#31688=DIRECTION('ref_axis',(1.,0.,0.));
#31689=DIRECTION('',(0.,0.,-1.));
#31690=DIRECTION('center_axis',(0.,0.,-1.));
#31691=DIRECTION('ref_axis',(1.,0.,0.));
#31692=DIRECTION('center_axis',(0.,0.,-1.));
#31693=DIRECTION('ref_axis',(1.,0.,0.));
#31694=DIRECTION('',(0.,0.,-1.));
#31695=DIRECTION('center_axis',(0.,0.,1.));
#31696=DIRECTION('ref_axis',(1.,0.,0.));
#31697=DIRECTION('center_axis',(0.,0.,-1.));
#31698=DIRECTION('ref_axis',(1.,0.,0.));
#31699=DIRECTION('center_axis',(0.,0.,-1.));
#31700=DIRECTION('ref_axis',(1.,0.,0.));
#31701=DIRECTION('',(0.,0.,-1.));
#31702=DIRECTION('center_axis',(0.,0.,1.));
#31703=DIRECTION('ref_axis',(1.,0.,0.));
#31704=DIRECTION('center_axis',(0.,0.,-1.));
#31705=DIRECTION('ref_axis',(1.,0.,0.));
#31706=DIRECTION('center_axis',(0.,0.,-1.));
#31707=DIRECTION('ref_axis',(1.,0.,0.));
#31708=DIRECTION('',(0.,0.,-1.));
#31709=DIRECTION('center_axis',(0.,0.,1.));
#31710=DIRECTION('ref_axis',(1.,0.,0.));
#31711=DIRECTION('center_axis',(0.,0.,1.));
#31712=DIRECTION('ref_axis',(1.,0.,0.));
#31713=DIRECTION('center_axis',(0.,0.,1.));
#31714=DIRECTION('ref_axis',(1.,0.,0.));
#31715=DIRECTION('center_axis',(0.,0.,1.));
#31716=DIRECTION('ref_axis',(1.,0.,0.));
#31717=DIRECTION('center_axis',(0.,0.,1.));
#31718=DIRECTION('ref_axis',(1.,0.,0.));
#31719=DIRECTION('center_axis',(0.,0.,1.));
#31720=DIRECTION('ref_axis',(1.,0.,0.));
#31721=DIRECTION('center_axis',(0.,0.,-1.));
#31722=DIRECTION('ref_axis',(1.,0.,0.));
#31723=DIRECTION('center_axis',(0.,0.,1.));
#31724=DIRECTION('ref_axis',(1.,0.,0.));
#31725=DIRECTION('',(0.,0.,-1.));
#31726=DIRECTION('center_axis',(0.,0.,1.));
#31727=DIRECTION('ref_axis',(1.,0.,0.));
#31728=DIRECTION('',(0.,0.,-1.));
#31729=DIRECTION('center_axis',(0.,0.,-1.));
#31730=DIRECTION('ref_axis',(1.,0.,0.));
#31731=DIRECTION('center_axis',(0.,0.,1.));
#31732=DIRECTION('ref_axis',(1.,0.,0.));
#31733=DIRECTION('',(0.,0.,-1.));
#31734=DIRECTION('center_axis',(0.,0.,1.));
#31735=DIRECTION('ref_axis',(1.,0.,0.));
#31736=DIRECTION('center_axis',(0.,0.,1.));
#31737=DIRECTION('ref_axis',(1.,0.,0.));
#31738=DIRECTION('center_axis',(0.,0.,1.));
#31739=DIRECTION('ref_axis',(1.,0.,0.));
#31740=DIRECTION('center_axis',(0.,0.,1.));
#31741=DIRECTION('ref_axis',(1.,0.,0.));
#31742=DIRECTION('center_axis',(0.,0.,1.));
#31743=DIRECTION('ref_axis',(1.,0.,0.));
#31744=DIRECTION('center_axis',(0.,0.,1.));
#31745=DIRECTION('ref_axis',(1.,0.,0.));
#31746=DIRECTION('center_axis',(0.,0.,-1.));
#31747=DIRECTION('ref_axis',(1.,0.,0.));
#31748=DIRECTION('center_axis',(0.,0.,1.));
#31749=DIRECTION('ref_axis',(1.,0.,0.));
#31750=DIRECTION('',(0.,0.,-1.));
#31751=DIRECTION('center_axis',(0.,0.,1.));
#31752=DIRECTION('ref_axis',(1.,0.,0.));
#31753=DIRECTION('',(0.,0.,-1.));
#31754=DIRECTION('center_axis',(0.,0.,-1.));
#31755=DIRECTION('ref_axis',(1.,0.,0.));
#31756=DIRECTION('center_axis',(0.,0.,1.));
#31757=DIRECTION('ref_axis',(1.,0.,0.));
#31758=DIRECTION('center_axis',(0.,0.,-1.));
#31759=DIRECTION('ref_axis',(1.,0.,0.));
#31760=DIRECTION('center_axis',(0.,0.,1.));
#31761=DIRECTION('ref_axis',(1.,0.,0.));
#31762=DIRECTION('',(0.,0.,-1.));
#31763=DIRECTION('center_axis',(0.,0.,1.));
#31764=DIRECTION('ref_axis',(1.,0.,0.));
#31765=DIRECTION('center_axis',(0.,0.,1.));
#31766=DIRECTION('ref_axis',(1.,0.,0.));
#31767=DIRECTION('',(0.,0.,-1.));
#31768=DIRECTION('center_axis',(0.,0.,-1.));
#31769=DIRECTION('ref_axis',(1.,0.,0.));
#31770=DIRECTION('center_axis',(0.,0.,1.));
#31771=DIRECTION('ref_axis',(1.,0.,0.));
#31772=DIRECTION('center_axis',(0.,0.,1.));
#31773=DIRECTION('ref_axis',(1.,0.,0.));
#31774=DIRECTION('',(0.,0.,-1.));
#31775=DIRECTION('center_axis',(0.,0.,1.));
#31776=DIRECTION('ref_axis',(1.,0.,0.));
#31777=DIRECTION('center_axis',(0.,0.,1.));
#31778=DIRECTION('ref_axis',(1.,0.,0.));
#31779=DIRECTION('center_axis',(0.,0.,1.));
#31780=DIRECTION('ref_axis',(1.,0.,0.));
#255772=CARTESIAN_POINT('',(0.,0.,0.));
#255773=CARTESIAN_POINT('Origin',(11.,-3.,98.));
#255774=CARTESIAN_POINT('',(7.41619848709566,-3.,86.));
#255775=CARTESIAN_POINT('',(7.41619848709566,-3.,98.));
#255776=CARTESIAN_POINT('',(7.41619848709566,-3.,78.));
#255777=CARTESIAN_POINT('',(5.,-3.,86.));
#255778=CARTESIAN_POINT('',(5.,-3.,86.));
#255779=CARTESIAN_POINT('',(5.,-3.,98.));
#255780=CARTESIAN_POINT('',(5.,-3.,98.));
#255781=CARTESIAN_POINT('',(5.,-3.,98.));
#255782=CARTESIAN_POINT('Origin',(8.,0.,98.));
#255783=CARTESIAN_POINT('',(7.41619848709566,3.,98.));
#255784=CARTESIAN_POINT('Origin',(0.,0.,98.));
#255785=CARTESIAN_POINT('',(5.,3.,98.));
#255786=CARTESIAN_POINT('',(5.,3.,98.));
#255787=CARTESIAN_POINT('',(11.,3.,98.));
#255788=CARTESIAN_POINT('Origin',(5.,3.,98.));
#255789=CARTESIAN_POINT('',(7.41619848709566,3.,86.));
#255790=CARTESIAN_POINT('',(7.41619848709566,3.,78.));
#255791=CARTESIAN_POINT('',(5.,3.,86.));
#255792=CARTESIAN_POINT('',(5.,3.,98.));
#255793=CARTESIAN_POINT('',(11.,3.,86.));
#255794=CARTESIAN_POINT('Origin',(5.,-3.,98.));
#255795=CARTESIAN_POINT('',(5.,3.,86.));
#255796=CARTESIAN_POINT('Origin',(8.,0.,86.));
#255797=CARTESIAN_POINT('Origin',(0.,0.,86.));
#255798=CARTESIAN_POINT('Origin',(0.,0.,100.5));
#255799=CARTESIAN_POINT('',(-7.,-8.57252759403147E-16,100.));
#255800=CARTESIAN_POINT('Origin',(0.,0.,100.));
#255801=CARTESIAN_POINT('',(-7.,-8.57252759403147E-16,101.));
#255802=CARTESIAN_POINT('',(-7.,-8.57252759403147E-16,100.5));
#255803=CARTESIAN_POINT('Origin',(0.,0.,101.));
#255804=CARTESIAN_POINT('Origin',(11.,0.,100.));
#255805=CARTESIAN_POINT('',(-8.,9.79717439317883E-16,100.));
#255806=CARTESIAN_POINT('Origin',(0.,0.,100.));
#255807=CARTESIAN_POINT('Origin',(7.,0.,101.));
#255808=CARTESIAN_POINT('',(-8.,-9.79717439317883E-16,101.));
#255809=CARTESIAN_POINT('Origin',(0.,0.,101.));
#255810=CARTESIAN_POINT('Origin',(0.,0.,78.));
#255811=CARTESIAN_POINT('',(-8.,-9.79717439317883E-16,113.));
#255812=CARTESIAN_POINT('Origin',(0.,0.,113.));
#255813=CARTESIAN_POINT('',(-8.,-9.79717439317883E-16,78.));
#255814=CARTESIAN_POINT('Origin',(0.,0.,76.5));
#255815=CARTESIAN_POINT('',(-15.,-1.83697019872103E-15,76.));
#255816=CARTESIAN_POINT('Origin',(0.,0.,76.));
#255817=CARTESIAN_POINT('',(-15.,-1.83697019872103E-15,77.));
#255818=CARTESIAN_POINT('',(-15.,-1.83697019872103E-15,76.5));
#255819=CARTESIAN_POINT('Origin',(0.,0.,77.));
#255820=CARTESIAN_POINT('Origin',(19.,0.,76.));
#255821=CARTESIAN_POINT('',(-16.,1.95943487863577E-15,76.));
#255822=CARTESIAN_POINT('Origin',(0.,0.,76.));
#255823=CARTESIAN_POINT('Origin',(15.,0.,77.));
#255824=CARTESIAN_POINT('',(-16.,-1.95943487863577E-15,77.));
#255825=CARTESIAN_POINT('Origin',(0.,0.,77.));
#255826=CARTESIAN_POINT('Origin',(0.,0.,54.));
#255827=CARTESIAN_POINT('',(-16.,-1.95943487863577E-15,78.));
#255828=CARTESIAN_POINT('Origin',(0.,0.,78.));
#255829=CARTESIAN_POINT('',(-16.,-1.95943487863577E-15,54.));
#255830=CARTESIAN_POINT('Origin',(-24.,41.5692193816531,50.));
#255831=CARTESIAN_POINT('',(-29.,41.5692193816531,54.));
#255832=CARTESIAN_POINT('Origin',(-24.,41.5692193816531,54.));
#255833=CARTESIAN_POINT('',(-29.,41.5692193816531,46.));
#255834=CARTESIAN_POINT('',(-29.,41.5692193816531,50.));
#255835=CARTESIAN_POINT('Origin',(-24.,41.5692193816531,46.));
#255836=CARTESIAN_POINT('Origin',(48.,0.,50.));
#255837=CARTESIAN_POINT('',(43.,6.12323399573677E-16,54.));
#255838=CARTESIAN_POINT('Origin',(48.,0.,54.));
#255839=CARTESIAN_POINT('',(43.,6.12323399573677E-16,46.));
#255840=CARTESIAN_POINT('',(43.,6.12323399573677E-16,50.));
#255841=CARTESIAN_POINT('Origin',(48.,0.,46.));
#255842=CARTESIAN_POINT('Origin',(-24.,-41.569219381653,50.));
#255843=CARTESIAN_POINT('',(-29.,-41.569219381653,54.));
#255844=CARTESIAN_POINT('Origin',(-24.,-41.569219381653,54.));
#255845=CARTESIAN_POINT('',(-29.,-41.569219381653,46.));
#255846=CARTESIAN_POINT('',(-29.,-41.569219381653,50.));
#255847=CARTESIAN_POINT('Origin',(-24.,-41.569219381653,46.));
#255848=CARTESIAN_POINT('Origin',(0.,0.,84.));
#255849=CARTESIAN_POINT('',(-11.,-1.34711147906209E-15,84.));
#255850=CARTESIAN_POINT('Origin',(0.,0.,84.));
#255851=CARTESIAN_POINT('',(-8.,-9.79717439317883E-16,84.));
#255852=CARTESIAN_POINT('Origin',(0.,0.,84.));
#255853=CARTESIAN_POINT('Origin',(0.,0.,82.));
#255854=CARTESIAN_POINT('',(-11.,-1.34711147906209E-15,82.));
#255855=CARTESIAN_POINT('Origin',(0.,0.,82.));
#255856=CARTESIAN_POINT('',(-8.,9.79717439317883E-16,82.));
#255857=CARTESIAN_POINT('Origin',(0.,0.,82.));
#255858=CARTESIAN_POINT('Origin',(0.,0.,82.));
#255859=CARTESIAN_POINT('',(-11.,-1.34711147906209E-15,82.));
#255860=CARTESIAN_POINT('Origin',(0.,0.,78.));
#255861=CARTESIAN_POINT('',(-8.,-9.79717439317883E-16,78.));
#255862=CARTESIAN_POINT('',(-8.,-9.79717439317883E-16,78.));
#255863=CARTESIAN_POINT('Origin',(0.,0.,78.));
#255864=CARTESIAN_POINT('Origin',(0.,0.,78.));
#255865=CARTESIAN_POINT('',(-8.,-9.79717439317883E-16,78.));
#255866=CARTESIAN_POINT('Origin',(0.,0.,113.));
#255867=CARTESIAN_POINT('Origin',(0.,0.,64.));
#255868=CARTESIAN_POINT('',(-20.,-2.44929359829471E-15,64.));
#255869=CARTESIAN_POINT('Origin',(0.,0.,64.));
#255870=CARTESIAN_POINT('',(-16.,-1.95943487863577E-15,64.));
#255871=CARTESIAN_POINT('Origin',(0.,0.,64.));
#255872=CARTESIAN_POINT('Origin',(0.,0.,62.));
#255873=CARTESIAN_POINT('',(-20.,-2.44929359829471E-15,62.));
#255874=CARTESIAN_POINT('Origin',(0.,0.,62.));
#255875=CARTESIAN_POINT('',(-16.,1.95943487863577E-15,62.));
#255876=CARTESIAN_POINT('Origin',(0.,0.,62.));
#255877=CARTESIAN_POINT('Origin',(0.,0.,62.));
#255878=CARTESIAN_POINT('',(-20.,-2.44929359829471E-15,62.));
#255879=CARTESIAN_POINT('Origin',(0.,0.,54.));
#255880=CARTESIAN_POINT('',(-16.,-1.95943487863577E-15,54.));
#255881=CARTESIAN_POINT('',(-16.,-1.95943487863577E-15,54.));
#255882=CARTESIAN_POINT('Origin',(0.,0.,54.));
#255883=CARTESIAN_POINT('Origin',(0.,0.,54.));
#255884=CARTESIAN_POINT('',(-12.,-1.46957615897682E-15,54.));
#255885=CARTESIAN_POINT('Origin',(0.,0.,54.));
#255886=CARTESIAN_POINT('Origin',(0.,0.,54.));
#255887=CARTESIAN_POINT('',(-16.,-1.95943487863577E-15,54.));
#255888=CARTESIAN_POINT('Origin',(0.,0.,78.));
#255889=CARTESIAN_POINT('Origin',(0.,0.,46.));
#255890=CARTESIAN_POINT('',(-12.,-1.46957615897682E-15,46.));
#255891=CARTESIAN_POINT('',(-12.,-1.46957615897682E-15,46.));
#255892=CARTESIAN_POINT('Origin',(0.,0.,46.));
#255893=CARTESIAN_POINT('Origin',(0.,0.,46.));
#255894=CARTESIAN_POINT('',(-70.,-8.57252759403147E-15,54.));
#255895=CARTESIAN_POINT('Origin',(0.,0.,54.));
#255896=CARTESIAN_POINT('',(-70.,-8.57252759403147E-15,46.));
#255897=CARTESIAN_POINT('',(-70.,-8.57252759403147E-15,46.));
#255898=CARTESIAN_POINT('Origin',(0.,0.,46.));
#255899=CARTESIAN_POINT('Origin',(0.,0.,54.));
#255900=CARTESIAN_POINT('Origin',(0.,0.,46.));
#259190=UNCERTAINTY_MEASURE_WITH_UNIT(LENGTH_MEASURE(0.01),#259225,
'DISTANCE_ACCURACY_VALUE',
'Maximum model space distance between geometric entities at asserted c
onnectivities');
#259202=UNCERTAINTY_MEASURE_WITH_UNIT(LENGTH_MEASURE(0.01),#259225,
'DISTANCE_ACCURACY_VALUE',
'Maximum model space distance between geometric entities at asserted c
onnectivities');
#259212=(
GEOMETRIC_REPRESENTATION_CONTEXT(3)
GLOBAL_UNCERTAINTY_ASSIGNED_CONTEXT((#259190))
GLOBAL_UNIT_ASSIGNED_CONTEXT((#259225,#259227,#259228))
REPRESENTATION_CONTEXT('','3D')
);
#259224=(
GEOMETRIC_REPRESENTATION_CONTEXT(3)
GLOBAL_UNCERTAINTY_ASSIGNED_CONTEXT((#259202))
GLOBAL_UNIT_ASSIGNED_CONTEXT((#259225,#259227,#259228))
REPRESENTATION_CONTEXT('','3D')
);
#259225=(
LENGTH_UNIT()
NAMED_UNIT(*)
SI_UNIT(.MILLI.,.METRE.)
);
#259227=(
NAMED_UNIT(*)
PLANE_ANGLE_UNIT()
SI_UNIT($,.RADIAN.)
);
#259228=(
NAMED_UNIT(*)
SI_UNIT($,.STERADIAN.)
SOLID_ANGLE_UNIT()
);
#259238=SHAPE_DEFINITION_REPRESENTATION(#259259,#259378);
#259259=PRODUCT_DEFINITION_SHAPE('',$,#259400);
#259378=SHAPE_REPRESENTATION('',(#27010),#259212);
#259390=PRODUCT_DEFINITION_CONTEXT('part definition',#259455,'design');
#259400=PRODUCT_DEFINITION('Carrier','Carrier',#259421,#259390);
#259421=PRODUCT_DEFINITION_FORMATION('',$,#259466);
#259455=APPLICATION_CONTEXT(
'Core Data for Automotive Mechanical Design Process');
#259456=PRODUCT_CONTEXT('part definition',#259455,'mechanical');
#259466=PRODUCT('Carrier','Carrier',$,(#259456));
#259486=PRESENTATION_STYLE_ASSIGNMENT((#259501));
#259501=SURFACE_STYLE_USAGE(.BOTH.,#259516);
#259516=SURFACE_SIDE_STYLE('',(#259531));
#259531=SURFACE_STYLE_FILL_AREA(#259546);
#259546=FILL_AREA_STYLE('Carrier sky blue',(#259561));
#259561=FILL_AREA_STYLE_COLOUR('Carrier sky blue',#259576);
#259576=COLOUR_RGB('Carrier sky blue',0.317647058823529,0.686274509803922,
0.890196078431372);
ENDSEC;
END-ISO-10303-21;
